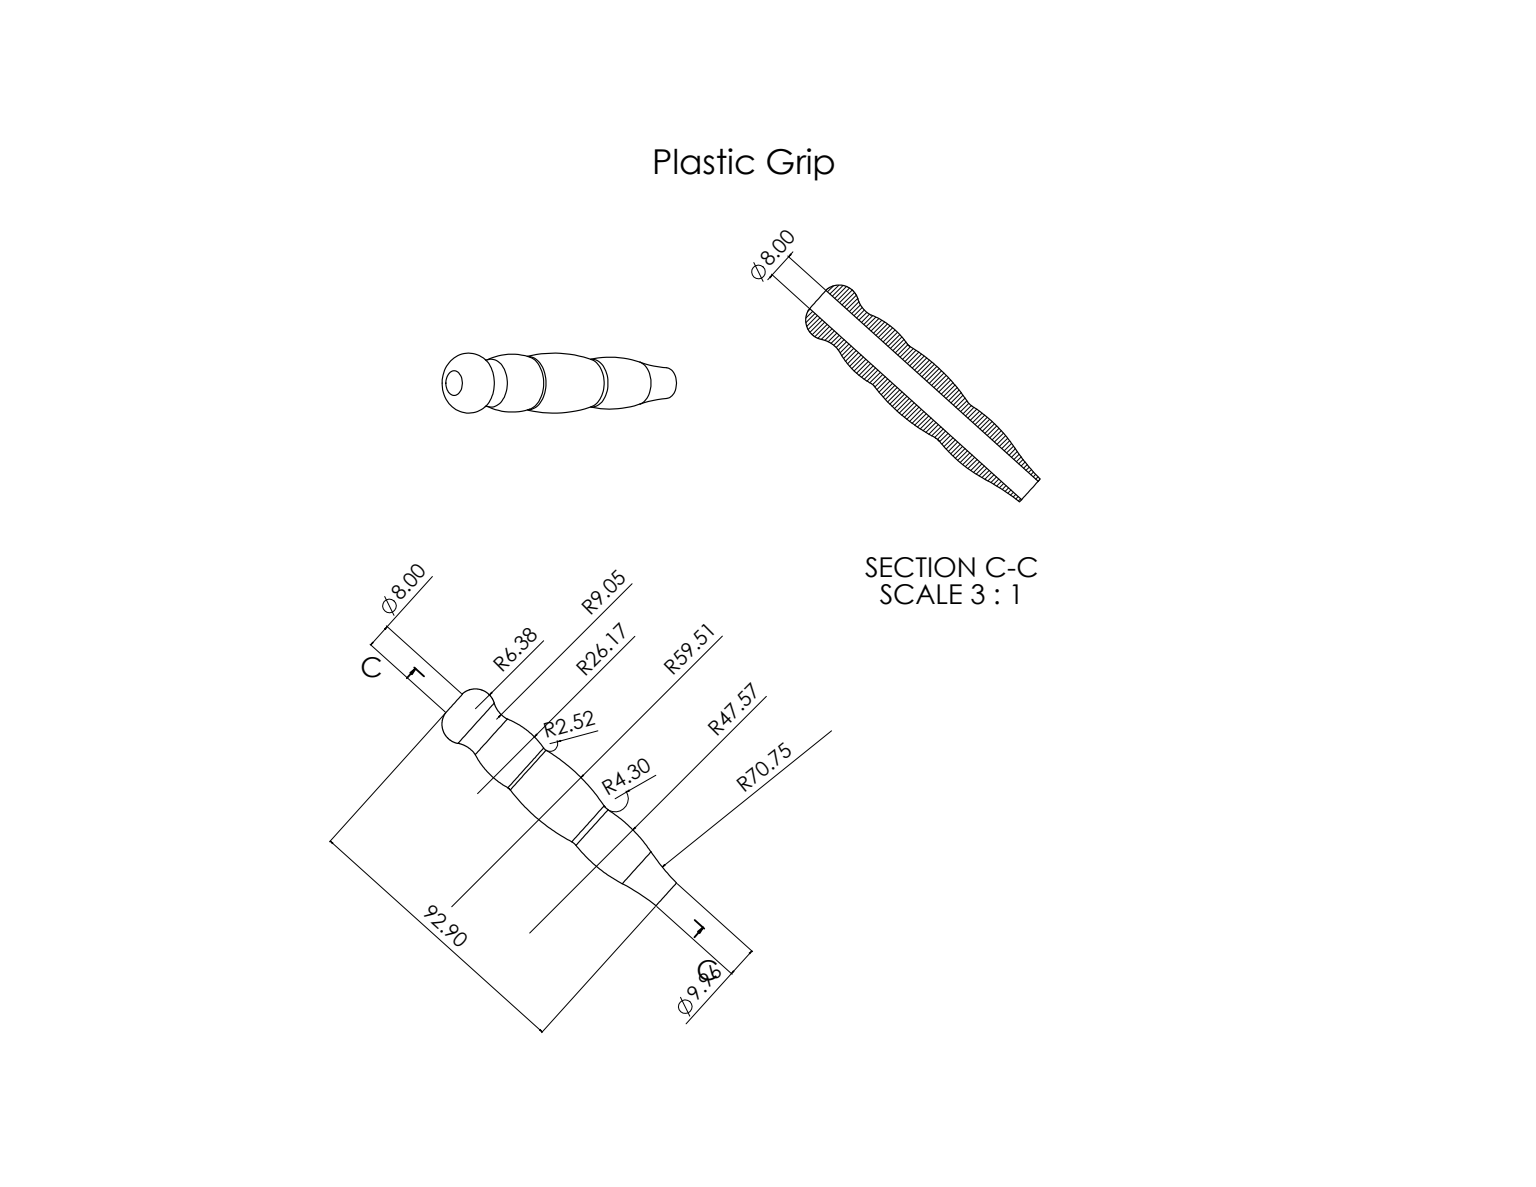
ISO-10303-21;
HEADER;
FILE_DESCRIPTION (('STEP AP214'),
    '1' );
FILE_NAME ('Plastic Grip.step',
    '2026-10-20T14:49:59',
    ( '' ),
    ( '' ),
    'SwSTEP 2.0',
    'SolidWorks 2025',
    '' );
FILE_SCHEMA (( 'AUTOMOTIVE_DESIGN' ));
ENDSEC;

DATA;
#4=DIRECTION ( 'NONE',  ( -0.6691306063588561281, -0.7431448254773960205, 0.000000000000000000 ) ) ;
#14=DIRECTION ( 'NONE',  ( -0.6691306063588562392, -0.7431448254773959095, 0.000000000000000000 ) ) ;
#16=DIRECTION ( 'NONE',  ( -0.6691306063588565722, -0.7431448254773957984, 0.000000000000000000 ) ) ;
#24=DIRECTION ( 'NONE',  ( 0.000000000000000000, -1.000000000000000000, -9.100899318238107179E-17 ) ) ;
#101=EDGE_CURVE ( 'NONE', #6753, #3816, #8421, .T. ) ;
#112=AXIS2_PLACEMENT_3D ( 'NONE', #10075, #7738, #3660 ) ;
#132=DIRECTION ( 'NONE',  ( -0.7431448254773957984, 0.6691306063588565722, -0.000000000000000000 ) ) ;
#158=CIRCLE ( 'NONE', #4883, 4.982234098198590644 ) ;
#169=EDGE_CURVE ( 'NONE', #490, #9911, #7578, .T. ) ;
#177=DIRECTION ( 'NONE',  ( -8.194486552889013533E-17, -9.100899318238110877E-17, 1.000000000000000000 ) ) ;
#179=DIRECTION ( 'NONE',  ( -0.6691306063588574604, -0.7431448254773949103, 0.000000000000000000 ) ) ;
#183=CARTESIAN_POINT ( 'NONE',  ( -147.2606667696710474, 253.8574007319445229, 0.000000000000000000 ) ) ;
#197=DIRECTION ( 'NONE',  ( -0.6691306063588565722, -0.7431448254773959095, 0.000000000000000000 ) ) ;
#213=DIRECTION ( 'NONE',  ( -0.7431448254773957984, 0.6691306063588565722, -0.000000000000000000 ) ) ;
#237=DIRECTION ( 'NONE',  ( -0.7431448254773957984, 0.6691306063588565722, -0.000000000000000000 ) ) ;
#238=ADVANCED_FACE ( 'NONE', ( #290 ), #4855, .T. ) ;
#241=CARTESIAN_POINT ( 'NONE',  ( -142.3328939341254795, 249.4204141414382434, 0.000000000000000000 ) ) ;
#247=PRODUCT_DEFINITION_FORMATION_WITH_SPECIFIED_SOURCE ( 'ANY', '', #7048, .NOT_KNOWN. ) ;
#290=FACE_OUTER_BOUND ( 'NONE', #9585, .T. ) ;
#292=AXIS2_PLACEMENT_3D ( 'NONE', #10403, #6319, #9565 ) ;
#299=DIRECTION ( 'NONE',  ( -8.194486552889013533E-17, -9.100899318238110877E-17, 1.000000000000000000 ) ) ;
#306=ORIENTED_EDGE ( 'NONE', *, *, #8464, .F. ) ;
#341=CARTESIAN_POINT ( 'NONE',  ( -152.9991366487805067, 270.9406871569508439, 1.084494555200859138E-15 ) ) ;
#347=EDGE_LOOP ( 'NONE', ( #2435, #5782, #9896, #402 ) ) ;
#357=EDGE_CURVE ( 'NONE', #2439, #4517, #2671, .T. ) ;
#394=TOROIDAL_SURFACE ( 'NONE', #3944, 11.15107097094592881, 2.515249034521771510 ) ;
#402=ORIENTED_EDGE ( 'NONE', *, *, #1707, .F. ) ;
#405=DIRECTION ( 'NONE',  ( -0.7431448254773957984, 0.6691306063588565722, -0.000000000000000000 ) ) ;
#430=EDGE_CURVE ( 'NONE', #1386, #2425, #494, .T. ) ;
#442=EDGE_LOOP ( 'NONE', ( #9473, #3806 ) ) ;
#486=ORIENTED_EDGE ( 'NONE', *, *, #169, .T. ) ;
#490=VERTEX_POINT ( 'NONE', #341 ) ;
#494=LINE ( 'NONE', #10247, #6224 ) ;
#551=TOROIDAL_SURFACE ( 'NONE', #6465, 16.62298474266377468, 9.050254677131421843 ) ;
#556=EDGE_CURVE ( 'NONE', #9911, #2425, #6732, .T. ) ;
#562=ORIENTED_EDGE ( 'NONE', *, *, #7593, .F. ) ;
#566=SHAPE_DEFINITION_REPRESENTATION ( #3920, #9697 ) ;
#576=CARTESIAN_POINT ( 'NONE',  ( -89.14744694221916177, 254.1708682956268603, 0.000000000000000000 ) ) ;
#585=ORIENTED_EDGE ( 'NONE', *, *, #5654, .F. ) ;
#591=DIRECTION ( 'NONE',  ( 0.000000000000000000, -1.000000000000000000, -9.100899318238089922E-17 ) ) ;
#594=AXIS2_PLACEMENT_3D ( 'NONE', #3166, #9596, #3115 ) ;
#617=CIRCLE ( 'NONE', #1964, 4.295524112943372330 ) ;
#642=DIRECTION ( 'NONE',  ( 0.000000000000000000, -0.000000000000000000, -1.000000000000000000 ) ) ;
#651=AXIS2_PLACEMENT_3D ( 'NONE', #10194, #3565, #8546 ) ;
#680=CARTESIAN_POINT ( 'NONE',  ( -166.0794662972351716, 270.8019239353934040, 0.000000000000000000 ) ) ;
#687=PRODUCT_DEFINITION ( 'UNKNOWN', '', #247, #5891 ) ;
#702=DIRECTION ( 'NONE',  ( -0.7431448254773957984, 0.6691306063588565722, -0.000000000000000000 ) ) ;
#728=TOROIDAL_SURFACE ( 'NONE', #9364, 3.377784142883041074, 6.382478589986769535 ) ;
#745=EDGE_CURVE ( 'NONE', #2342, #2439, #3018, .T. ) ;
#756=AXIS2_PLACEMENT_3D ( 'NONE', #4002, #6747, #591 ) ;
#765=DIRECTION ( 'NONE',  ( -0.6691306063588566833, -0.7431448254773957984, 0.000000000000000000 ) ) ;
#768=ORIENTED_EDGE ( 'NONE', *, *, #5611, .F. ) ;
#778=FACE_OUTER_BOUND ( 'NONE', #5546, .T. ) ;
#787=CIRCLE ( 'NONE', #8916, 8.635821936424155965 ) ;
#794=ORIENTED_EDGE ( 'NONE', *, *, #1876, .T. ) ;
#802=FACE_OUTER_BOUND ( 'NONE', #3369, .T. ) ;
#810=CARTESIAN_POINT ( 'NONE',  ( -142.3328939341254795, 249.4204141414382434, 0.000000000000000000 ) ) ;
#833=EDGE_CURVE ( 'NONE', #8917, #6087, #10133, .T. ) ;
#858=ORIENTED_EDGE ( 'NONE', *, *, #2768, .F. ) ;
#888=DIRECTION ( 'NONE',  ( -0.7431448254773957984, 0.6691306063588565722, -0.000000000000000000 ) ) ;
#889=AXIS2_PLACEMENT_3D ( 'NONE', #4773, #8859, #2296 ) ;
#891=CIRCLE ( 'NONE', #3260, 9.050254677131441383 ) ;
#892=DIRECTION ( 'NONE',  ( -0.7431448254773957984, 0.6691306063588565722, -0.000000000000000000 ) ) ;
#902=DIRECTION ( 'NONE',  ( -0.6691306063588566833, -0.7431448254773955764, 0.000000000000000000 ) ) ;
#961=AXIS2_PLACEMENT_3D ( 'NONE', #4774, #8012, #3991 ) ;
#1016=ORIENTED_EDGE ( 'NONE', *, *, #2108, .T. ) ;
#1025=DIRECTION ( 'NONE',  ( -0.6691306063588565722, -0.7431448254773957984, 0.000000000000000000 ) ) ;
#1052=EDGE_CURVE ( 'NONE', #9925, #6648, #8435, .T. ) ;
#1062=CARTESIAN_POINT ( 'NONE',  ( -163.4029438717997209, 273.7745032373030085, 4.898587196589436495E-16 ) ) ;
#1092=ORIENTED_EDGE ( 'NONE', *, *, #2031, .F. ) ;
#1096=AXIS2_PLACEMENT_3D ( 'NONE', #8801, #3977, #8692 ) ;
#1110=EDGE_CURVE ( 'NONE', #2425, #9911, #6741, .T. ) ;
#1124=EDGE_CURVE ( 'NONE', #4793, #490, #1337, .T. ) ;
#1138=CARTESIAN_POINT ( 'NONE',  ( -155.4728935706336301, 261.2517229562222951, 0.000000000000000000 ) ) ;
#1151=ORIENTED_EDGE ( 'NONE', *, *, #4635, .T. ) ;
#1156=DIRECTION ( 'NONE',  ( -0.7431448254773957984, 0.6691306063588565722, -0.000000000000000000 ) ) ;
#1165=CIRCLE ( 'NONE', #7936, 8.635821936424155965 ) ;
#1184=DIRECTION ( 'NONE',  ( -0.6691306063588565722, -0.7431448254773956874, 0.000000000000000000 ) ) ;
#1194=CARTESIAN_POINT ( 'NONE',  ( -117.2684580747526581, 237.4318902223653254, 9.628383344360778382E-16 ) ) ;
#1215=MECHANICAL_DESIGN_GEOMETRIC_PRESENTATION_REPRESENTATION('',(#9163),#6451);
#1241=DIRECTION ( 'NONE',  ( -8.194486552889013533E-17, -9.100899318238110877E-17, 1.000000000000000000 ) ) ;
#1246=DIRECTION ( 'NONE',  ( -0.6691306063588565722, -0.7431448254773957984, 0.000000000000000000 ) ) ;
#1259=ADVANCED_FACE ( 'NONE', ( #9754 ), #6405, .T. ) ;
#1272=ORIENTED_EDGE ( 'NONE', *, *, #10189, .T. ) ;
#1281=AXIS2_PLACEMENT_3D ( 'NONE', #3694, #405, #1246 ) ;
#1296=TOROIDAL_SURFACE ( 'NONE', #961, 12.02085523418795177, 4.295524112943378547 ) ;
#1337=CIRCLE ( 'NONE', #2348, 8.855570079111213744 ) ;
#1386=VERTEX_POINT ( 'NONE', #3486 ) ;
#1402=DIRECTION ( 'NONE',  ( -0.6691306063588565722, -0.7431448254773956874, 0.000000000000000000 ) ) ;
#1424=DIRECTION ( 'NONE',  ( -0.7431448254773957984, 0.6691306063588565722, -0.000000000000000000 ) ) ;
#1441=CIRCLE ( 'NONE', #6166, 7.794205612481196255 ) ;
#1448=DIRECTION ( 'NONE',  ( -0.7431448254773957984, 0.6691306063588565722, -0.000000000000000000 ) ) ;
#1452=AXIS2_PLACEMENT_3D ( 'NONE', #8678, #4652, #9540 ) ;
#1490=EDGE_CURVE ( 'NONE', #490, #4793, #9756, .T. ) ;
#1520=PRODUCT_CONTEXT ( 'NONE', #1525, 'mechanical' ) ;
#1525=APPLICATION_CONTEXT ( 'automotive_design' ) ;
#1531=DIRECTION ( 'NONE',  ( -0.6691306063588601249, -0.7431448254773928008, 0.000000000000000000 ) ) ;
#1544=ORIENTED_EDGE ( 'NONE', *, *, #5654, .T. ) ;
#1550=DIRECTION ( 'NONE',  ( -0.6691306063588565722, -0.7431448254773957984, 0.000000000000000000 ) ) ;
#1555=EDGE_LOOP ( 'NONE', ( #6042, #8592, #8206, #858 ) ) ;
#1573=DIRECTION ( 'NONE',  ( 0.000000000000000000, -0.000000000000000000, -1.000000000000000000 ) ) ;
#1583=CIRCLE ( 'NONE', #3443, 4.000000000000007994 ) ;
#1586=DIRECTION ( 'NONE',  ( -0.7431448254773957984, 0.6691306063588565722, -0.000000000000000000 ) ) ;
#1590=ORIENTED_EDGE ( 'NONE', *, *, #3868, .F. ) ;
#1601=DIRECTION ( 'NONE',  ( -0.7431448254773957984, 0.6691306063588565722, -0.000000000000000000 ) ) ;
#1607=ORIENTED_EDGE ( 'NONE', *, *, #3884, .T. ) ;
#1617=ORIENTED_EDGE ( 'NONE', *, *, #9294, .F. ) ;
#1620=DIRECTION ( 'NONE',  ( -0.7431448254773957984, 0.6691306063588565722, -0.000000000000000000 ) ) ;
#1629=ORIENTED_EDGE ( 'NONE', *, *, #8965, .F. ) ;
#1638=DIRECTION ( 'NONE',  ( -0.6691306063588564612, -0.7431448254773956874, 0.000000000000000000 ) ) ;
#1655=DIRECTION ( 'NONE',  ( -0.7431448254773957984, 0.6691306063588565722, -0.000000000000000000 ) ) ;
#1702=CARTESIAN_POINT ( 'NONE',  ( -142.3328939341254795, 249.4204141414382434, 0.000000000000000000 ) ) ;
#1707=EDGE_CURVE ( 'NONE', #2362, #6151, #617, .T. ) ;
#1745=ADVANCED_FACE ( 'NONE', ( #9238 ), #6205, .F. ) ;
#1754=TOROIDAL_SURFACE ( 'NONE', #7008, 75.59748767972220662, 70.74985237403969052 ) ;
#1758=DIRECTION ( 'NONE',  ( -0.7431448254773957984, 0.6691306063588565722, -0.000000000000000000 ) ) ;
#1760=AXIS2_PLACEMENT_3D ( 'NONE', #680, #3111, #2163 ) ;
#1767=DIRECTION ( 'NONE',  ( -8.194486552889013533E-17, -9.100899318238110877E-17, 1.000000000000000000 ) ) ;
#1770=ORIENTED_EDGE ( 'NONE', *, *, #1110, .T. ) ;
#1813=ORIENTED_EDGE ( 'NONE', *, *, #2108, .F. ) ;
#1818=VECTOR ( 'NONE', #8221, 1000.000000000000114 ) ;
#1821=DIRECTION ( 'NONE',  ( -0.7431448254773957984, 0.6691306063588565722, -0.000000000000000000 ) ) ;
#1822=CARTESIAN_POINT ( 'NONE',  ( -153.9940972124336156, 259.9202087346060921, 0.000000000000000000 ) ) ;
#1830=AXIS2_PLACEMENT_3D ( 'NONE', #3609, #9278, #9979 ) ;
#1839=CARTESIAN_POINT ( 'NONE',  ( -148.5890485138274357, 243.3411686721859724, 0.000000000000000000 ) ) ;
#1841=ORIENTED_EDGE ( 'NONE', *, *, #10189, .F. ) ;
#1876=EDGE_CURVE ( 'NONE', #2362, #4450, #4513, .T. ) ;
#1949=EDGE_CURVE ( 'NONE', #1386, #1994, #5353, .T. ) ;
#1951=DIRECTION ( 'NONE',  ( -0.7431448254773957984, 0.6691306063588565722, -0.000000000000000000 ) ) ;
#1964=AXIS2_PLACEMENT_3D ( 'NONE', #5307, #5253, #4469 ) ;
#1980=CARTESIAN_POINT ( 'NONE',  ( -126.4085176256957084, 224.6061440934676909, 0.000000000000000000 ) ) ;
#1994=VERTEX_POINT ( 'NONE', #10129 ) ;
#2023=ORIENTED_EDGE ( 'NONE', *, *, #6467, .F. ) ;
#2031=EDGE_CURVE ( 'NONE', #5603, #4869, #3842, .T. ) ;
#2034=CARTESIAN_POINT ( 'NONE',  ( -134.8713710537857935, 257.7072748320279061, 1.365612337163390183E-15 ) ) ;
#2039=CARTESIAN_POINT ( 'NONE',  ( -163.4029438717996641, 273.7745032373030654, 4.898587196589562712E-16 ) ) ;
#2041=CIRCLE ( 'NONE', #6279, 7.785108809001807906 ) ;
#2065=FACE_OUTER_BOUND ( 'NONE', #5158, .T. ) ;
#2075=DIRECTION ( 'NONE',  ( -0.7431448254773956874, 0.6691306063588564612, -0.000000000000000000 ) ) ;
#2080=ADVANCED_FACE ( 'NONE', ( #4069 ), #6880, .T. ) ;
#2084=CIRCLE ( 'NONE', #7345, 2.515249034521771510 ) ;
#2108=EDGE_CURVE ( 'NONE', #4793, #8917, #10105, .T. ) ;
#2135=CIRCLE ( 'NONE', #8753, 7.862171649053781408 ) ;
#2153=EDGE_CURVE ( 'NONE', #2439, #2342, #3160, .T. ) ;
#2156=ORIENTED_EDGE ( 'NONE', *, *, #5857, .T. ) ;
#2159=ORIENTED_EDGE ( 'NONE', *, *, #9094, .F. ) ;
#2163=DIRECTION ( 'NONE',  ( -0.6691306063588601249, -0.7431448254773928008, 0.000000000000000000 ) ) ;
#2176=AXIS2_PLACEMENT_3D ( 'NONE', #2955, #1586, #8257 ) ;
#2188=DIRECTION ( 'NONE',  ( -8.194486552889013533E-17, -9.100899318238110877E-17, 1.000000000000000000 ) ) ;
#2194=CARTESIAN_POINT ( 'NONE',  ( -121.7299640054770578, 230.8694527092982867, 0.000000000000000000 ) ) ;
#2209=VERTEX_POINT ( 'NONE', #5968 ) ;
#2250=CARTESIAN_POINT ( 'NONE',  ( -111.3540224549888933, 212.1074838665961124, 0.000000000000000000 ) ) ;
#2252=DIRECTION ( 'NONE',  ( -0.7431448254773957984, 0.6691306063588565722, -0.000000000000000000 ) ) ;
#2271=CYLINDRICAL_SURFACE ( 'NONE', #1760, 4.000000000000016875 ) ;
#2296=DIRECTION ( 'NONE',  ( -0.6691306063588566833, -0.7431448254773956874, 0.000000000000000000 ) ) ;
#2342=VERTEX_POINT ( 'NONE', #1839 ) ;
#2346=CARTESIAN_POINT ( 'NONE',  ( -133.6038276124207300, 241.5607275224312787, 0.000000000000000000 ) ) ;
#2348=AXIS2_PLACEMENT_3D ( 'NONE', #6563, #3221, #8145 ) ;
#2350=FACE_OUTER_BOUND ( 'NONE', #6872, .T. ) ;
#2362=VERTEX_POINT ( 'NONE', #2842 ) ;
#2379=DIRECTION ( 'NONE',  ( -0.7431448254773957984, 0.6691306063588565722, -0.000000000000000000 ) ) ;
#2425=VERTEX_POINT ( 'NONE', #6929 ) ;
#2428=CARTESIAN_POINT ( 'NONE',  ( -115.3226892516804583, 225.1003166080523954, 0.000000000000000000 ) ) ;
#2432=DIRECTION ( 'NONE',  ( -0.6691306063588580155, -0.7431448254773944662, 0.000000000000000000 ) ) ;
#2435=ORIENTED_EDGE ( 'NONE', *, *, #2550, .F. ) ;
#2439=VERTEX_POINT ( 'NONE', #5384 ) ;
#2490=TOROIDAL_SURFACE ( 'NONE', #3682, 75.59748767972220662, 70.74985237403969052 ) ;
#2539=ORIENTED_EDGE ( 'NONE', *, *, #4294, .T. ) ;
#2550=EDGE_CURVE ( 'NONE', #4450, #2362, #7596, .T. ) ;
#2604=ORIENTED_EDGE ( 'NONE', *, *, #9461, .T. ) ;
#2609=EDGE_CURVE ( 'NONE', #4517, #4542, #1165, .T. ) ;
#2650=CIRCLE ( 'NONE', #6207, 70.74985237403969052 ) ;
#2651=ORIENTED_EDGE ( 'NONE', *, *, #2153, .F. ) ;
#2671=CIRCLE ( 'NONE', #651, 2.515249034521771510 ) ;
#2703=CARTESIAN_POINT ( 'NONE',  ( -141.9789400531797412, 249.1017126355397977, 0.000000000000000000 ) ) ;
#2721=FACE_OUTER_BOUND ( 'NONE', #6822, .T. ) ;
#2724=( NAMED_UNIT ( * ) PLANE_ANGLE_UNIT ( ) SI_UNIT ( $, .RADIAN. ) );
#2733=ORIENTED_EDGE ( 'NONE', *, *, #5857, .F. ) ;
#2734=AXIS2_PLACEMENT_3D ( 'NONE', #3821, #642, #9493 ) ;
#2744=CARTESIAN_POINT ( 'NONE',  ( -126.8992195029584025, 225.1284128614458950, 0.000000000000000000 ) ) ;
#2752=CIRCLE ( 'NONE', #889, 7.785108809001807906 ) ;
#2767=FACE_OUTER_BOUND ( 'NONE', #347, .T. ) ;
#2768=EDGE_CURVE ( 'NONE', #4517, #4943, #9289, .T. ) ;
#2772=CIRCLE ( 'NONE', #8702, 26.17065043502059396 ) ;
#2779=ADVANCED_FACE ( 'NONE', ( #2721 ), #5394, .F. ) ;
#2807=EDGE_LOOP ( 'NONE', ( #1841, #3283, #8792, #3496 ) ) ;
#2829=DIRECTION ( 'NONE',  ( -0.6691306063588566833, -0.7431448254773957984, 0.000000000000000000 ) ) ;
#2839=ORIENTED_EDGE ( 'NONE', *, *, #8183, .F. ) ;
#2842=CARTESIAN_POINT ( 'NONE',  ( -116.5607085079957130, 236.6104925571506783, 9.460802029985586576E-16 ) ) ;
#2882=EDGE_CURVE ( 'NONE', #6578, #8917, #9644, .T. ) ;
#2914=AXIS2_PLACEMENT_3D ( 'NONE', #5840, #237, #4308 ) ;
#2935=DIRECTION ( 'NONE',  ( -0.7431448254773957984, 0.6691306063588565722, -0.000000000000000000 ) ) ;
#2944=EDGE_CURVE ( 'NONE', #3816, #6753, #158, .T. ) ;
#2954=FACE_OUTER_BOUND ( 'NONE', #9451, .T. ) ;
#2955=CARTESIAN_POINT ( 'NONE',  ( -166.0794662972351716, 270.8019239353934040, 0.000000000000000000 ) ) ;
#2959=FACE_OUTER_BOUND ( 'NONE', #10440, .T. ) ;
#2965=ORIENTED_EDGE ( 'NONE', *, *, #2768, .T. ) ;
#2972=DIRECTION ( 'NONE',  ( -0.6691306063588565722, -0.7431448254773957984, 0.000000000000000000 ) ) ;
#2993=ADVANCED_FACE ( 'NONE', ( #7227, #8864 ), #4926, .F. ) ;
#2999=DIRECTION ( 'NONE',  ( -0.7431448254773957984, 0.6691306063588565722, -0.000000000000000000 ) ) ;
#3009=DIRECTION ( 'NONE',  ( -1.000000000000000000, 0.000000000000000000, 0.000000000000000000 ) ) ;
#3011=ADVANCED_FACE ( 'NONE', ( #8067 ), #7604, .F. ) ;
#3018=CIRCLE ( 'NONE', #4369, 8.703944320672444945 ) ;
#3032=AXIS2_PLACEMENT_3D ( 'NONE', #810, #7276, #16 ) ;
#3053=CARTESIAN_POINT ( 'NONE',  ( -121.7299640054770578, 230.8694527092982867, 0.000000000000000000 ) ) ;
#3085=DIRECTION ( 'NONE',  ( -0.7431448254773957984, 0.6691306063588565722, -0.000000000000000000 ) ) ;
#3088=DIRECTION ( 'NONE',  ( -0.6691306063588565722, -0.7431448254773957984, 0.000000000000000000 ) ) ;
#3101=FACE_OUTER_BOUND ( 'NONE', #7591, .T. ) ;
#3111=DIRECTION ( 'NONE',  ( -0.7431448254773957984, 0.6691306063588565722, -0.000000000000000000 ) ) ;
#3115=DIRECTION ( 'NONE',  ( -0.6691306063588566833, -0.7431448254773957984, 0.000000000000000000 ) ) ;
#3125=EDGE_CURVE ( 'NONE', #4793, #2425, #7435, .T. ) ;
#3143=CARTESIAN_POINT ( 'NONE',  ( -150.4057481100919915, 266.8793581191597468, 9.273919635561124944E-16 ) ) ;
#3150=CARTESIAN_POINT ( 'NONE',  ( -160.5400390311752403, 255.6240877932848150, 0.000000000000000000 ) ) ;
#3155=ORIENTED_EDGE ( 'NONE', *, *, #2550, .T. ) ;
#3160=CIRCLE ( 'NONE', #7070, 8.703944320672444945 ) ;
#3166=CARTESIAN_POINT ( 'NONE',  ( -155.4728935706336301, 261.2517229562222951, 0.000000000000000000 ) ) ;
#3179=CARTESIAN_POINT ( 'NONE',  ( -153.9940972124336156, 259.9202087346060921, 0.000000000000000000 ) ) ;
#3184=EDGE_LOOP ( 'NONE', ( #7189, #4392, #7724, #2651 ) ) ;
#3221=DIRECTION ( 'NONE',  ( -0.7431448254773957984, 0.6691306063588565722, -0.000000000000000000 ) ) ;
#3242=AXIS2_PLACEMENT_3D ( 'NONE', #2428, #888, #5757 ) ;
#3247=DIRECTION ( 'NONE',  ( -0.6691306063588566833, -0.7431448254773957984, 0.000000000000000000 ) ) ;
#3248=CIRCLE ( 'NONE', #9348, 59.51479730733485951 ) ;
#3257=TOROIDAL_SURFACE ( 'NONE', #9703, 12.02085523418795177, 4.295524112943378547 ) ;
#3260=AXIS2_PLACEMENT_3D ( 'NONE', #8498, #299, #6697 ) ;
#3262=EDGE_LOOP ( 'NONE', ( #6618, #5581 ) ) ;
#3279=DIRECTION ( 'NONE',  ( -0.7431448254773957984, 0.6691306063588565722, -0.000000000000000000 ) ) ;
#3283=ORIENTED_EDGE ( 'NONE', *, *, #5473, .T. ) ;
#3287=ORIENTED_EDGE ( 'NONE', *, *, #3125, .F. ) ;
#3369=EDGE_LOOP ( 'NONE', ( #6942, #1272, #1590, #5013 ) ) ;
#3392=ORIENTED_EDGE ( 'NONE', *, *, #5271, .F. ) ;
#3398=AXIS2_PLACEMENT_3D ( 'NONE', #7312, #9814, #4287 ) ;
#3443=AXIS2_PLACEMENT_3D ( 'NONE', #4909, #892, #2432 ) ;
#3455=AXIS2_PLACEMENT_3D ( 'NONE', #4155, #1767, #24 ) ;
#3457=UNCERTAINTY_MEASURE_WITH_UNIT (LENGTH_MEASURE( 1.000000000000000082E-05 ), #7613, 'distance_accuracy_value', 'NONE');
#3461=ADVANCED_FACE ( 'NONE', ( #8938 ), #2490, .F. ) ;
#3466=CARTESIAN_POINT ( 'NONE',  ( -161.3589532509997468, 266.5515548974023545, 0.000000000000000000 ) ) ;
#3473=ORIENTED_EDGE ( 'NONE', *, *, #8527, .T. ) ;
#3486=CARTESIAN_POINT ( 'NONE',  ( -99.71820871057254010, 205.6674483012464520, 0.000000000000000000 ) ) ;
#3496=ORIENTED_EDGE ( 'NONE', *, *, #7879, .F. ) ;
#3500=ORIENTED_EDGE ( 'NONE', *, *, #4372, .T. ) ;
#3507=DIRECTION ( 'NONE',  ( 0.000000000000000000, -0.000000000000000000, -1.000000000000000000 ) ) ;
#3530=( LENGTH_UNIT ( ) NAMED_UNIT ( * ) SI_UNIT ( .MILLI., .METRE. ) );
#3565=DIRECTION ( 'NONE',  ( -8.194486552889013533E-17, -9.100899318238110877E-17, 1.000000000000000000 ) ) ;
#3575=DIRECTION ( 'NONE',  ( -0.7431448254773957984, 0.6691306063588565722, -0.000000000000000000 ) ) ;
#3583=ORIENTED_EDGE ( 'NONE', *, *, #745, .T. ) ;
#3609=CARTESIAN_POINT ( 'NONE',  ( -166.5958414309862690, 248.8984378607219980, 0.000000000000000000 ) ) ;
#3616=ORIENTED_EDGE ( 'NONE', *, *, #169, .F. ) ;
#3653=DIRECTION ( 'NONE',  ( -0.6691306063588566833, -0.7431448254773956874, 0.000000000000000000 ) ) ;
#3660=DIRECTION ( 'NONE',  ( -0.6691306063588580155, -0.7431448254773944662, 0.000000000000000000 ) ) ;
#3682=AXIS2_PLACEMENT_3D ( 'NONE', #4950, #1620, #197 ) ;
#3688=AXIS2_PLACEMENT_3D ( 'NONE', #2703, #5089, #4142 ) ;
#3694=CARTESIAN_POINT ( 'NONE',  ( -115.3226892516804583, 225.1003166080523954, 0.000000000000000000 ) ) ;
#3763=CARTESIAN_POINT ( 'NONE',  ( -122.5292777575814114, 231.5891580443559121, 0.000000000000000000 ) ) ;
#3798=CARTESIAN_POINT ( 'NONE',  ( -155.4728935706336301, 261.2517229562222951, 0.000000000000000000 ) ) ;
#3806=ORIENTED_EDGE ( 'NONE', *, *, #101, .F. ) ;
#3809=DIRECTION ( 'NONE',  ( -0.6691306063588565722, -0.7431448254773957984, 0.000000000000000000 ) ) ;
#3816=VERTEX_POINT ( 'NONE', #6114 ) ;
#3821=CARTESIAN_POINT ( 'NONE',  ( -129.7734861572812974, 221.9362163441986411, 0.000000000000000000 ) ) ;
#3833=CARTESIAN_POINT ( 'NONE',  ( -166.8975519277663295, 204.5843006325352746, -6.093437144708294610E-15 ) ) ;
#3842=CIRCLE ( 'NONE', #8059, 7.862171649053781408 ) ;
#3861=ORIENTED_EDGE ( 'NONE', *, *, #7879, .T. ) ;
#3866=DIRECTION ( 'NONE',  ( 0.000000000000000000, -0.000000000000000000, -1.000000000000000000 ) ) ;
#3868=EDGE_CURVE ( 'NONE', #9316, #4943, #5198, .T. ) ;
#3872=CARTESIAN_POINT ( 'NONE',  ( -113.6864418536728465, 239.8026890743979322, 1.472130188556198457E-15 ) ) ;
#3884=EDGE_CURVE ( 'NONE', #1994, #9911, #9173, .T. ) ;
#3909=EDGE_LOOP ( 'NONE', ( #3616, #7241, #7180, #9613 ) ) ;
#3916=DIRECTION ( 'NONE',  ( -1.000000000000000000, 0.000000000000000000, 0.000000000000000000 ) ) ;
#3920=PRODUCT_DEFINITION_SHAPE ( 'NONE', 'NONE',  #687 ) ;
#3933=ORIENTED_EDGE ( 'NONE', *, *, #8965, .T. ) ;
#3944=AXIS2_PLACEMENT_3D ( 'NONE', #10404, #1448, #1550 ) ;
#3977=DIRECTION ( 'NONE',  ( -0.7431448254773957984, 0.6691306063588565722, -0.000000000000000000 ) ) ;
#3991=DIRECTION ( 'NONE',  ( -0.6691306063588565722, -0.7431448254773956874, 0.000000000000000000 ) ) ;
#4002=CARTESIAN_POINT ( 'NONE',  ( -144.3499457102809913, 273.6050080517225638, 2.035728505737848743E-15 ) ) ;
#4069=FACE_OUTER_BOUND ( 'NONE', #2807, .T. ) ;
#4142=DIRECTION ( 'NONE',  ( -0.6691306063588549069, -0.7431448254773971307, 0.000000000000000000 ) ) ;
#4146=CARTESIAN_POINT ( 'NONE',  ( -93.70792096198771048, 212.3425490925493762, 0.000000000000000000 ) ) ;
#4155=CARTESIAN_POINT ( 'NONE',  ( -158.4738950245593117, 241.4038491004292837, -2.052251677020569255E-15 ) ) ;
#4201=AXIS2_PLACEMENT_3D ( 'NONE', #6196, #5452, #4606 ) ;
#4258=FACE_OUTER_BOUND ( 'NONE', #1555, .T. ) ;
#4260=AXIS2_PLACEMENT_3D ( 'NONE', #2194, #6219, #1402 ) ;
#4287=DIRECTION ( 'NONE',  ( -1.000000000000000000, 0.000000000000000000, 0.000000000000000000 ) ) ;
#4294=EDGE_CURVE ( 'NONE', #2342, #4542, #5981, .T. ) ;
#4298=ORIENTED_EDGE ( 'NONE', *, *, #1052, .T. ) ;
#4302=CARTESIAN_POINT ( 'NONE',  ( -163.6191320026764231, 264.0413720900392036, 0.000000000000000000 ) ) ;
#4304=ORIENTED_EDGE ( 'NONE', *, *, #5557, .T. ) ;
#4308=DIRECTION ( 'NONE',  ( -0.6691306063588562392, -0.7431448254773960205, 0.000000000000000000 ) ) ;
#4352=EDGE_LOOP ( 'NONE', ( #2539, #4304, #8852, #4892 ) ) ;
#4358=AXIS2_PLACEMENT_3D ( 'NONE', #3872, #8887, #7837 ) ;
#4369=AXIS2_PLACEMENT_3D ( 'NONE', #4872, #6622, #902 ) ;
#4372=EDGE_CURVE ( 'NONE', #8917, #6578, #5664, .T. ) ;
#4391=AXIS2_PLACEMENT_3D ( 'NONE', #2034, #1241, #8499 ) ;
#4392=ORIENTED_EDGE ( 'NONE', *, *, #2609, .T. ) ;
#4410=ORIENTED_EDGE ( 'NONE', *, *, #9461, .F. ) ;
#4450=VERTEX_POINT ( 'NONE', #2744 ) ;
#4469=DIRECTION ( 'NONE',  ( 0.000000000000000000, -1.000000000000000000, -9.100899318238123202E-17 ) ) ;
#4490=ORIENTED_EDGE ( 'NONE', *, *, #2882, .T. ) ;
#4496=CARTESIAN_POINT ( 'NONE',  ( -148.1113867028520872, 243.0027477556404563, 0.000000000000000000 ) ) ;
#4500=DIRECTION ( 'NONE',  ( -0.6691306063588562392, -0.7431448254773959095, 0.000000000000000000 ) ) ;
#4509=DIRECTION ( 'NONE',  ( -0.7431448254773957984, 0.6691306063588565722, -0.000000000000000000 ) ) ;
#4513=CIRCLE ( 'NONE', #292, 7.725331121244574994 ) ;
#4517=VERTEX_POINT ( 'NONE', #8419 ) ;
#4522=DIRECTION ( 'NONE',  ( -0.7431448254773957984, 0.6691306063588565722, -0.000000000000000000 ) ) ;
#4542=VERTEX_POINT ( 'NONE', #4496 ) ;
#4545=CARTESIAN_POINT ( 'NONE',  ( -155.4728935706336301, 261.2517229562222951, 0.000000000000000000 ) ) ;
#4558=DIRECTION ( 'NONE',  ( -0.7431448254773957984, 0.6691306063588565722, -0.000000000000000000 ) ) ;
#4590=ADVANCED_FACE ( 'NONE', ( #5495 ), #10281, .F. ) ;
#4596=CARTESIAN_POINT ( 'NONE',  ( -149.7944168144651655, 241.1335534508485807, 0.000000000000000000 ) ) ;
#4599=CARTESIAN_POINT ( 'NONE',  ( -141.4979315611417690, 196.0297649204779589, -4.790608351577442020E-15 ) ) ;
#4601=AXIS2_PLACEMENT_3D ( 'NONE', #8586, #5983, #5928 ) ;
#4606=DIRECTION ( 'NONE',  ( -0.6691306063588562392, -0.7431448254773960205, 0.000000000000000000 ) ) ;
#4635=EDGE_CURVE ( 'NONE', #9925, #6753, #10417, .T. ) ;
#4648=CARTESIAN_POINT ( 'NONE',  ( -158.9246696254695337, 264.3597160760069187, 0.000000000000000000 ) ) ;
#4652=DIRECTION ( 'NONE',  ( -8.194486552889013533E-17, -9.100899318238110877E-17, 1.000000000000000000 ) ) ;
#4681=CIRCLE ( 'NONE', #5852, 7.794205612481196255 ) ;
#4729=ORIENTED_EDGE ( 'NONE', *, *, #9294, .T. ) ;
#4739=DIRECTION ( 'NONE',  ( -0.7431448254773957984, 0.6691306063588565722, -0.000000000000000000 ) ) ;
#4753=ORIENTED_EDGE ( 'NONE', *, *, #1110, .F. ) ;
#4770=DIRECTION ( 'NONE',  ( 0.000000000000000000, -1.000000000000000000, -9.100899318238112109E-17 ) ) ;
#4773=CARTESIAN_POINT ( 'NONE',  ( -121.1992630477586346, 230.3916074206559017, 0.000000000000000000 ) ) ;
#4774=CARTESIAN_POINT ( 'NONE',  ( -121.7299640054770578, 230.8694527092982867, 0.000000000000000000 ) ) ;
#4793=VERTEX_POINT ( 'NONE', #9744 ) ;
#4803=TOROIDAL_SURFACE ( 'NONE', #6163, 11.15107097094592881, 2.515249034521771510 ) ;
#4845=ORIENTED_EDGE ( 'NONE', *, *, #1124, .T. ) ;
#4855=TOROIDAL_SURFACE ( 'NONE', #6220, -16.75790667520975674, 26.17065043502059041 ) ;
#4856=CARTESIAN_POINT ( 'NONE',  ( -166.5958414309862690, 248.8984378607219980, 0.000000000000000000 ) ) ;
#4869=VERTEX_POINT ( 'NONE', #1194 ) ;
#4872=CARTESIAN_POINT ( 'NONE',  ( -142.7649729728221359, 249.8094598553370531, 0.000000000000000000 ) ) ;
#4881=ADVANCED_FACE ( 'NONE', ( #7661 ), #9760, .T. ) ;
#4882=ORIENTED_EDGE ( 'NONE', *, *, #430, .T. ) ;
#4883=AXIS2_PLACEMENT_3D ( 'NONE', #9831, #1758, #179 ) ;
#4892=ORIENTED_EDGE ( 'NONE', *, *, #745, .F. ) ;
#4909=CARTESIAN_POINT ( 'NONE',  ( -97.04168628513710360, 208.6400276031560281, 0.000000000000000000 ) ) ;
#4926=PLANE ( 'NONE',  #9120 ) ;
#4943=VERTEX_POINT ( 'NONE', #9633 ) ;
#4950=CARTESIAN_POINT ( 'NONE',  ( -93.80004353141508489, 205.7212393575359783, 0.000000000000000000 ) ) ;
#4953=CIRCLE ( 'NONE', #5292, 8.681329343575942659 ) ;
#4967=CARTESIAN_POINT ( 'NONE',  ( -155.4728935706336301, 261.2517229562222951, 0.000000000000000000 ) ) ;
#4975=CIRCLE ( 'NONE', #3455, 26.17065043502059396 ) ;
#4979=ORIENTED_EDGE ( 'NONE', *, *, #9094, .T. ) ;
#5013=ORIENTED_EDGE ( 'NONE', *, *, #7178, .F. ) ;
#5052=AXIS2_PLACEMENT_3D ( 'NONE', #1138, #3575, #6111 ) ;
#5089=DIRECTION ( 'NONE',  ( -0.7431448254773957984, 0.6691306063588565722, -0.000000000000000000 ) ) ;
#5158=EDGE_LOOP ( 'NONE', ( #4845, #486, #4753, #3287 ) ) ;
#5168=ORIENTED_EDGE ( 'NONE', *, *, #1949, .F. ) ;
#5198=CIRCLE ( 'NONE', #3688, 8.681329343575942659 ) ;
#5240=ORIENTED_EDGE ( 'NONE', *, *, #5611, .T. ) ;
#5253=DIRECTION ( 'NONE',  ( -8.194486552889013533E-17, -9.100899318238110877E-17, 1.000000000000000000 ) ) ;
#5255=DIRECTION ( 'NONE',  ( -0.7431448254773957984, 0.6691306063588565722, -0.000000000000000000 ) ) ;
#5262=TOROIDAL_SURFACE ( 'NONE', #4260, 12.02085523418795177, 4.295524112943378547 ) ;
#5271=EDGE_CURVE ( 'NONE', #2209, #6087, #4681, .T. ) ;
#5292=AXIS2_PLACEMENT_3D ( 'NONE', #6949, #4558, #6038 ) ;
#5293=ORIENTED_EDGE ( 'NONE', *, *, #9517, .F. ) ;
#5295=CIRCLE ( 'NONE', #4358, 4.295524112943372330 ) ;
#5307=CARTESIAN_POINT ( 'NONE',  ( -113.6864418536728465, 239.8026890743979322, 1.472130188556198457E-15 ) ) ;
#5313=TOROIDAL_SURFACE ( 'NONE', #5650, 3.377784142883041074, 6.382478589986769535 ) ;
#5318=CIRCLE ( 'NONE', #756, 9.050254677131441383 ) ;
#5333=CARTESIAN_POINT ( 'NONE',  ( -100.3101032970751305, 278.5371544123273111, 0.000000000000000000 ) ) ;
#5353=CIRCLE ( 'NONE', #112, 4.000000000000007994 ) ;
#5372=ORIENTED_EDGE ( 'NONE', *, *, #556, .T. ) ;
#5384=CARTESIAN_POINT ( 'NONE',  ( -136.9408974318168646, 256.2777510384881339, 1.065925755226830171E-15 ) ) ;
#5394=TOROIDAL_SURFACE ( 'NONE', #8783, 16.62298474266377468, 9.050254677131421843 ) ;
#5414=CARTESIAN_POINT ( 'NONE',  ( -166.0794662972351716, 270.8019239353934040, 0.000000000000000000 ) ) ;
#5452=DIRECTION ( 'NONE',  ( -0.7431448254773957984, 0.6691306063588565722, -0.000000000000000000 ) ) ;
#5473=EDGE_CURVE ( 'NONE', #4869, #5603, #2135, .T. ) ;
#5477=DIRECTION ( 'NONE',  ( -0.6691306063588574604, -0.7431448254773949103, 0.000000000000000000 ) ) ;
#5495=FACE_OUTER_BOUND ( 'NONE', #9273, .T. ) ;
#5502=DIRECTION ( 'NONE',  ( -0.6691306063588566833, -0.7431448254773955764, 0.000000000000000000 ) ) ;
#5519=FACE_OUTER_BOUND ( 'NONE', #4352, .T. ) ;
#5537=AXIS2_PLACEMENT_3D ( 'NONE', #7080, #7230, #6330 ) ;
#5545=CARTESIAN_POINT ( 'NONE',  ( -142.3328939341254795, 249.4204141414382434, 0.000000000000000000 ) ) ;
#5546=EDGE_LOOP ( 'NONE', ( #5571, #4979, #8645, #9724 ) ) ;
#5549=DIRECTION ( 'NONE',  ( -0.7431448254773957984, 0.6691306063588565722, -0.000000000000000000 ) ) ;
#5557=EDGE_CURVE ( 'NONE', #4542, #4517, #787, .T. ) ;
#5571=ORIENTED_EDGE ( 'NONE', *, *, #2882, .F. ) ;
#5581=ORIENTED_EDGE ( 'NONE', *, *, #8183, .T. ) ;
#5582=CARTESIAN_POINT ( 'NONE',  ( -97.04168628513711781, 208.6400276031560566, 0.000000000000000000 ) ) ;
#5584=ADVANCED_FACE ( 'NONE', ( #8809 ), #1296, .F. ) ;
#5591=ORIENTED_EDGE ( 'NONE', *, *, #3884, .F. ) ;
#5603=VERTEX_POINT ( 'NONE', #7638 ) ;
#5611=EDGE_CURVE ( 'NONE', #9925, #6151, #7564, .T. ) ;
#5650=AXIS2_PLACEMENT_3D ( 'NONE', #3466, #7495, #1025 ) ;
#5654=EDGE_CURVE ( 'NONE', #6648, #3816, #2650, .T. ) ;
#5663=ORIENTED_EDGE ( 'NONE', *, *, #1490, .F. ) ;
#5664=CIRCLE ( 'NONE', #8720, 7.572730065532343069 ) ;
#5712=ORIENTED_EDGE ( 'NONE', *, *, #1052, .F. ) ;
#5757=DIRECTION ( 'NONE',  ( -0.6691306063588565722, -0.7431448254773957984, 0.000000000000000000 ) ) ;
#5759=FACE_OUTER_BOUND ( 'NONE', #9367, .T. ) ;
#5779=AXIS2_PLACEMENT_3D ( 'NONE', #3833, #2188, #4770 ) ;
#5782=ORIENTED_EDGE ( 'NONE', *, *, #6775, .T. ) ;
#5802=ADVANCED_FACE ( 'NONE', ( #778 ), #8025, .F. ) ;
#5822=ORIENTED_EDGE ( 'NONE', *, *, #4635, .F. ) ;
#5840=CARTESIAN_POINT ( 'NONE',  ( -106.6701082104768687, 217.3094976449379203, 0.000000000000000000 ) ) ;
#5852=AXIS2_PLACEMENT_3D ( 'NONE', #1822, #5255, #9241 ) ;
#5857=EDGE_CURVE ( 'NONE', #4869, #2362, #5295, .T. ) ;
#5869=DIRECTION ( 'NONE',  ( -1.000000000000000000, 0.000000000000000000, 0.000000000000000000 ) ) ;
#5891=PRODUCT_DEFINITION_CONTEXT ( 'detailed design', #10047, 'design' ) ;
#5928=DIRECTION ( 'NONE',  ( 1.000000000000000000, 0.000000000000000000, 0.000000000000000000 ) ) ;
#5932=CIRCLE ( 'NONE', #3398, 4.295524112943372330 ) ;
#5934=DIRECTION ( 'NONE',  ( -1.000000000000000000, 0.000000000000000000, 0.000000000000000000 ) ) ;
#5953=TOROIDAL_SURFACE ( 'NONE', #10032, 16.62298474266377468, 9.050254677131421843 ) ;
#5960=ORIENTED_EDGE ( 'NONE', *, *, #1707, .T. ) ;
#5968=CARTESIAN_POINT ( 'NONE',  ( -148.7787556848684858, 265.7124323042283436, 9.545148955221437884E-16 ) ) ;
#5981=CIRCLE ( 'NONE', #10413, 2.515249034521771510 ) ;
#5983=DIRECTION ( 'NONE',  ( 0.000000000000000000, 0.000000000000000000, 1.000000000000000000 ) ) ;
#5997=DIRECTION ( 'NONE',  ( -0.7431448254773957984, 0.6691306063588565722, -0.000000000000000000 ) ) ;
#6000=TOROIDAL_SURFACE ( 'NONE', #1096, 11.15107097094592881, 2.515249034521771510 ) ;
#6021=DIRECTION ( 'NONE',  ( -0.6691306063588564612, -0.7431448254773957984, 0.000000000000000000 ) ) ;
#6038=DIRECTION ( 'NONE',  ( -0.6691306063588549069, -0.7431448254773971307, 0.000000000000000000 ) ) ;
#6042=ORIENTED_EDGE ( 'NONE', *, *, #5557, .F. ) ;
#6047=ORIENTED_EDGE ( 'NONE', *, *, #7593, .T. ) ;
#6074=AXIS2_PLACEMENT_3D ( 'NONE', #4302, #8147, #9107 ) ;
#6087=VERTEX_POINT ( 'NONE', #9313 ) ;
#6111=DIRECTION ( 'NONE',  ( -0.6691306063588564612, -0.7431448254773956874, 0.000000000000000000 ) ) ;
#6114=CARTESIAN_POINT ( 'NONE',  ( -100.3754516082865393, 204.9375061137627370, 0.000000000000000000 ) ) ;
#6151=VERTEX_POINT ( 'NONE', #6385 ) ;
#6158=CARTESIAN_POINT ( 'NONE',  ( -121.7299640054770578, 230.8694527092982867, 0.000000000000000000 ) ) ;
#6163=AXIS2_PLACEMENT_3D ( 'NONE', #241, #1821, #2972 ) ;
#6166=AXIS2_PLACEMENT_3D ( 'NONE', #3179, #2379, #4 ) ;
#6196=CARTESIAN_POINT ( 'NONE',  ( -106.6701082104768687, 217.3094976449379203, 0.000000000000000000 ) ) ;
#6205=TOROIDAL_SURFACE ( 'NONE', #6710, 12.02085523418795177, 4.295524112943378547 ) ;
#6207=AXIS2_PLACEMENT_3D ( 'NONE', #9433, #3507, #5934 ) ;
#6219=DIRECTION ( 'NONE',  ( -0.7431448254773957984, 0.6691306063588565722, -0.000000000000000000 ) ) ;
#6220=AXIS2_PLACEMENT_3D ( 'NONE', #183, #132, #6638 ) ;
#6224=VECTOR ( 'NONE', #2075, 1000.000000000000114 ) ;
#6247=ADVANCED_FACE ( 'NONE', ( #3101 ), #551, .F. ) ;
#6265=DIRECTION ( 'NONE',  ( -0.6691306063588601249, -0.7431448254773928008, 0.000000000000000000 ) ) ;
#6279=AXIS2_PLACEMENT_3D ( 'NONE', #10125, #1951, #3653 ) ;
#6282=DIRECTION ( 'NONE',  ( -0.7431448254773957984, 0.6691306063588565722, -0.000000000000000000 ) ) ;
#6287=DIRECTION ( 'NONE',  ( -0.6691306063588547959, -0.7431448254773973527, 0.000000000000000000 ) ) ;
#6288=DIRECTION ( 'NONE',  ( -0.7431448254773957984, 0.6691306063588565722, -0.000000000000000000 ) ) ;
#6298=CARTESIAN_POINT ( 'NONE',  ( -142.7649729728221359, 249.8094598553370531, 0.000000000000000000 ) ) ;
#6319=DIRECTION ( 'NONE',  ( -0.7431448254773957984, 0.6691306063588565722, -0.000000000000000000 ) ) ;
#6330=DIRECTION ( 'NONE',  ( 0.000000000000000000, -1.000000000000000000, -9.100899318238137994E-17 ) ) ;
#6385=CARTESIAN_POINT ( 'NONE',  ( -115.9900084698215608, 236.1770707478440841, 9.534008583957946635E-16 ) ) ;
#6400=CARTESIAN_POINT ( 'NONE',  ( -133.6038276124207300, 241.5607275224312787, 0.000000000000000000 ) ) ;
#6405=TOROIDAL_SURFACE ( 'NONE', #7764, -16.75790667520975674, 26.17065043502059041 ) ;
#6451=( GEOMETRIC_REPRESENTATION_CONTEXT ( 3 ) GLOBAL_UNCERTAINTY_ASSIGNED_CONTEXT ( ( #3457 ) ) GLOBAL_UNIT_ASSIGNED_CONTEXT ( ( #7613, #7561, #10106 ) ) REPRESENTATION_CONTEXT ( 'NONE', 'WORKASPACE' ) );
#6465=AXIS2_PLACEMENT_3D ( 'NONE', #3798, #2999, #765 ) ;
#6467=EDGE_CURVE ( 'NONE', #490, #6578, #891, .T. ) ;
#6480=DIRECTION ( 'NONE',  ( 0.000000000000000000, -0.000000000000000000, -1.000000000000000000 ) ) ;
#6524=VERTEX_POINT ( 'NONE', #1980 ) ;
#6563=CARTESIAN_POINT ( 'NONE',  ( -158.9246696254695337, 264.3597160760069187, 0.000000000000000000 ) ) ;
#6578=VERTEX_POINT ( 'NONE', #3143 ) ;
#6618=ORIENTED_EDGE ( 'NONE', *, *, #1949, .T. ) ;
#6622=DIRECTION ( 'NONE',  ( -0.7431448254773957984, 0.6691306063588565722, -0.000000000000000000 ) ) ;
#6638=DIRECTION ( 'NONE',  ( -0.6691306063588564612, -0.7431448254773957984, 0.000000000000000000 ) ) ;
#6648=VERTEX_POINT ( 'NONE', #2250 ) ;
#6697=DIRECTION ( 'NONE',  ( 0.000000000000000000, -1.000000000000000000, -9.100899318238089922E-17 ) ) ;
#6702=ADVANCED_FACE ( 'NONE', ( #2350 ), #5262, .F. ) ;
#6706=( NAMED_UNIT ( * ) SI_UNIT ( $, .STERADIAN. ) SOLID_ANGLE_UNIT ( ) );
#6710=AXIS2_PLACEMENT_3D ( 'NONE', #6909, #5997, #7646 ) ;
#6732=CIRCLE ( 'NONE', #8254, 4.000000000000016875 ) ;
#6741=CIRCLE ( 'NONE', #2176, 4.000000000000016875 ) ;
#6747=DIRECTION ( 'NONE',  ( -8.194486552889013533E-17, -9.100899318238110877E-17, 1.000000000000000000 ) ) ;
#6750=ORIENTED_EDGE ( 'NONE', *, *, #5473, .F. ) ;
#6753=VERTEX_POINT ( 'NONE', #8796 ) ;
#6756=SHAPE_REPRESENTATION_RELATIONSHIP ( 'NONE' , 'NONE' ,  #9697, #9745 ) ;
#6775=EDGE_CURVE ( 'NONE', #4450, #6524, #6799, .T. ) ;
#6799=CIRCLE ( 'NONE', #2734, 4.295524112943372330 ) ;
#6814=TOROIDAL_SURFACE ( 'NONE', #9541, -49.75669024694125397, 59.51479730733485951 ) ;
#6822=EDGE_LOOP ( 'NONE', ( #1016, #3500, #2023, #8555 ) ) ;
#6837=ADVANCED_FACE ( 'NONE', ( #9440 ), #7814, .T. ) ;
#6872=EDGE_LOOP ( 'NONE', ( #8288, #5960, #6047, #7479 ) ) ;
#6880=TOROIDAL_SURFACE ( 'NONE', #9602, -49.75669024694125397, 59.51479730733485951 ) ;
#6909=CARTESIAN_POINT ( 'NONE',  ( -121.7299640054770578, 230.8694527092982867, 0.000000000000000000 ) ) ;
#6929=CARTESIAN_POINT ( 'NONE',  ( -168.7559887226705087, 267.8293446334839700, 0.000000000000000000 ) ) ;
#6934=CARTESIAN_POINT ( 'NONE',  ( -147.2606667696710474, 253.8574007319445229, 0.000000000000000000 ) ) ;
#6942=ORIENTED_EDGE ( 'NONE', *, *, #2031, .T. ) ;
#6949=CARTESIAN_POINT ( 'NONE',  ( -141.9789400531797412, 249.1017126355397977, 0.000000000000000000 ) ) ;
#7008=AXIS2_PLACEMENT_3D ( 'NONE', #9054, #3279, #7308 ) ;
#7034=ORIENTED_EDGE ( 'NONE', *, *, #2609, .F. ) ;
#7048=PRODUCT ( 'Plastic Grip', 'Plastic Grip', '', ( #1520 ) ) ;
#7060=CARTESIAN_POINT ( 'NONE',  ( -147.7878832208476183, 242.6502276555962396, 0.000000000000000000 ) ) ;
#7070=AXIS2_PLACEMENT_3D ( 'NONE', #6298, #10438, #5502 ) ;
#7077=AXIS2_PLACEMENT_3D ( 'NONE', #5582, #2252, #5477 ) ;
#7080=CARTESIAN_POINT ( 'NONE',  ( -159.0987744993230706, 269.0617377047655054, 4.136592538792403018E-16 ) ) ;
#7091=DIRECTION ( 'NONE',  ( -0.6691306063588553510, -0.7431448254773969087, 0.000000000000000000 ) ) ;
#7101=CARTESIAN_POINT ( 'NONE',  ( -166.0794662972351716, 270.8019239353934040, 0.000000000000000000 ) ) ;
#7167=ADVANCED_FACE ( 'NONE', ( #2954 ), #5953, .F. ) ;
#7178=EDGE_CURVE ( 'NONE', #5603, #9316, #3248, .T. ) ;
#7180=ORIENTED_EDGE ( 'NONE', *, *, #3125, .T. ) ;
#7189=ORIENTED_EDGE ( 'NONE', *, *, #357, .T. ) ;
#7198=DIRECTION ( 'NONE',  ( -1.000000000000000000, 0.000000000000000000, 0.000000000000000000 ) ) ;
#7216=EDGE_LOOP ( 'NONE', ( #7034, #2965, #3861, #306 ) ) ;
#7227=FACE_OUTER_BOUND ( 'NONE', #442, .T. ) ;
#7230=DIRECTION ( 'NONE',  ( -8.194486552889013533E-17, -9.100899318238110877E-17, 1.000000000000000000 ) ) ;
#7236=CLOSED_SHELL ( 'NONE', ( #1745, #7616, #2779, #7167, #3011, #5584, #4590, #8245, #4881, #6702, #7607, #9277, #1259, #5802, #7918, #9095, #6247, #238, #9111, #2080, #7410, #6837, #3461, #2993, #8538 ) ) ;
#7237=ORIENTED_EDGE ( 'NONE', *, *, #7301, .F. ) ;
#7241=ORIENTED_EDGE ( 'NONE', *, *, #1490, .T. ) ;
#7276=DIRECTION ( 'NONE',  ( -0.7431448254773957984, 0.6691306063588565722, -0.000000000000000000 ) ) ;
#7301=EDGE_CURVE ( 'NONE', #6648, #9925, #7486, .T. ) ;
#7308=DIRECTION ( 'NONE',  ( -0.6691306063588565722, -0.7431448254773959095, 0.000000000000000000 ) ) ;
#7312=CARTESIAN_POINT ( 'NONE',  ( -129.7734861572812974, 221.9362163441986411, 0.000000000000000000 ) ) ;
#7345=AXIS2_PLACEMENT_3D ( 'NONE', #4596, #1573, #7198 ) ;
#7354=ORIENTED_EDGE ( 'NONE', *, *, #833, .T. ) ;
#7410=ADVANCED_FACE ( 'NONE', ( #2767 ), #3257, .F. ) ;
#7432=DIRECTION ( 'NONE',  ( -0.6691306063588560171, -0.7431448254773961315, 0.000000000000000000 ) ) ;
#7433=ORIENTED_EDGE ( 'NONE', *, *, #7301, .T. ) ;
#7435=CIRCLE ( 'NONE', #6074, 6.382478589986778417 ) ;
#7479=ORIENTED_EDGE ( 'NONE', *, *, #6775, .F. ) ;
#7486=CIRCLE ( 'NONE', #2914, 7.000000000000016875 ) ;
#7495=DIRECTION ( 'NONE',  ( -0.7431448254773957984, 0.6691306063588565722, -0.000000000000000000 ) ) ;
#7561=( NAMED_UNIT ( * ) PLANE_ANGLE_UNIT ( ) SI_UNIT ( $, .RADIAN. ) );
#7564=CIRCLE ( 'NONE', #8241, 47.56532671630425568 ) ;
#7578=CIRCLE ( 'NONE', #5537, 6.382478589986750883 ) ;
#7586=CARTESIAN_POINT ( 'NONE',  ( -161.3589532509997468, 266.5515548974023545, 0.000000000000000000 ) ) ;
#7591=EDGE_LOOP ( 'NONE', ( #9394, #7354, #4729, #2159 ) ) ;
#7593=EDGE_CURVE ( 'NONE', #6151, #6524, #2752, .T. ) ;
#7596=CIRCLE ( 'NONE', #8946, 7.725331121244574994 ) ;
#7604=TOROIDAL_SURFACE ( 'NONE', #3032, 11.15107097094592881, 2.515249034521771510 ) ;
#7607=ADVANCED_FACE ( 'NONE', ( #802 ), #6814, .T. ) ;
#7613=( LENGTH_UNIT ( ) NAMED_UNIT ( * ) SI_UNIT ( .MILLI., .METRE. ) );
#7616=ADVANCED_FACE ( 'NONE', ( #5519 ), #394, .F. ) ;
#7638=CARTESIAN_POINT ( 'NONE',  ( -127.7900974404101930, 225.7464258663465557, 0.000000000000000000 ) ) ;
#7646=DIRECTION ( 'NONE',  ( -0.6691306063588565722, -0.7431448254773956874, 0.000000000000000000 ) ) ;
#7661=FACE_OUTER_BOUND ( 'NONE', #10437, .T. ) ;
#7683=CIRCLE ( 'NONE', #8531, 47.56532671630425568 ) ;
#7696=ORIENTED_EDGE ( 'NONE', *, *, #8449, .T. ) ;
#7724=ORIENTED_EDGE ( 'NONE', *, *, #4294, .F. ) ;
#7738=DIRECTION ( 'NONE',  ( -0.7431448254773957984, 0.6691306063588565722, -0.000000000000000000 ) ) ;
#7764=AXIS2_PLACEMENT_3D ( 'NONE', #6934, #1156, #6021 ) ;
#7814=TOROIDAL_SURFACE ( 'NONE', #3242, -39.11828581851394659, 47.56532671630426989 ) ;
#7837=DIRECTION ( 'NONE',  ( 0.000000000000000000, -1.000000000000000000, -9.100899318238123202E-17 ) ) ;
#7879=EDGE_CURVE ( 'NONE', #4943, #9316, #4953, .T. ) ;
#7918=ADVANCED_FACE ( 'NONE', ( #2065 ), #728, .T. ) ;
#7934=DIRECTION ( 'NONE',  ( -0.6691306063588560171, -0.7431448254773961315, 0.000000000000000000 ) ) ;
#7936=AXIS2_PLACEMENT_3D ( 'NONE', #5545, #4739, #7934 ) ;
#7940=DIRECTION ( 'NONE',  ( -1.000000000000000000, 0.000000000000000000, 0.000000000000000000 ) ) ;
#8012=DIRECTION ( 'NONE',  ( -0.7431448254773957984, 0.6691306063588565722, -0.000000000000000000 ) ) ;
#8025=TOROIDAL_SURFACE ( 'NONE', #594, 16.62298474266377468, 9.050254677131421843 ) ;
#8059=AXIS2_PLACEMENT_3D ( 'NONE', #3763, #9382, #4500 ) ;
#8067=FACE_OUTER_BOUND ( 'NONE', #3184, .T. ) ;
#8132=EDGE_LOOP ( 'NONE', ( #2156, #794, #4410, #6750 ) ) ;
#8142=DIRECTION ( 'NONE',  ( -0.7431448254773957984, 0.6691306063588565722, -0.000000000000000000 ) ) ;
#8145=DIRECTION ( 'NONE',  ( -0.6691306063588547959, -0.7431448254773973527, 0.000000000000000000 ) ) ;
#8147=DIRECTION ( 'NONE',  ( 0.000000000000000000, -0.000000000000000000, -1.000000000000000000 ) ) ;
#8149=CARTESIAN_POINT ( 'NONE',  ( -149.7944168144651655, 241.1335534508485807, 0.000000000000000000 ) ) ;
#8170=DIRECTION ( 'NONE',  ( -0.7431448254773957984, 0.6691306063588565722, 0.000000000000000000 ) ) ;
#8183=EDGE_CURVE ( 'NONE', #1994, #1386, #1583, .T. ) ;
#8206=ORIENTED_EDGE ( 'NONE', *, *, #3868, .T. ) ;
#8221=DIRECTION ( 'NONE',  ( -0.7431448254773956874, 0.6691306063588564612, -0.000000000000000000 ) ) ;
#8241=AXIS2_PLACEMENT_3D ( 'NONE', #4599, #177, #9229 ) ;
#8245=ADVANCED_FACE ( 'NONE', ( #5759 ), #1754, .F. ) ;
#8254=AXIS2_PLACEMENT_3D ( 'NONE', #5414, #3085, #6265 ) ;
#8257=DIRECTION ( 'NONE',  ( -0.6691306063588601249, -0.7431448254773928008, 0.000000000000000000 ) ) ;
#8287=FACE_OUTER_BOUND ( 'NONE', #3909, .T. ) ;
#8288=ORIENTED_EDGE ( 'NONE', *, *, #1876, .F. ) ;
#8322=CIRCLE ( 'NONE', #5779, 59.51479730733485951 ) ;
#8346=EDGE_LOOP ( 'NONE', ( #768, #4298, #7696, #562 ) ) ;
#8419=CARTESIAN_POINT ( 'NONE',  ( -136.5544011653988719, 255.8380805272360590, 1.057583169244835033E-15 ) ) ;
#8421=CIRCLE ( 'NONE', #7077, 4.982234098198590644 ) ;
#8429=DIRECTION ( 'NONE',  ( -0.6691306063588565722, -0.7431448254773957984, 0.000000000000000000 ) ) ;
#8435=CIRCLE ( 'NONE', #4201, 7.000000000000016875 ) ;
#8449=EDGE_CURVE ( 'NONE', #6648, #6524, #7683, .T. ) ;
#8464=EDGE_CURVE ( 'NONE', #4542, #9316, #2084, .T. ) ;
#8498=CARTESIAN_POINT ( 'NONE',  ( -144.3499457102809913, 273.6050080517225638, 2.035728505737848743E-15 ) ) ;
#8499=DIRECTION ( 'NONE',  ( 0.000000000000000000, -1.000000000000000000, -9.100899318238108411E-17 ) ) ;
#8527=EDGE_CURVE ( 'NONE', #2342, #6087, #2772, .T. ) ;
#8531=AXIS2_PLACEMENT_3D ( 'NONE', #576, #3866, #3916 ) ;
#8538=ADVANCED_FACE ( 'NONE', ( #2959 ), #2271, .F. ) ;
#8546=DIRECTION ( 'NONE',  ( 0.000000000000000000, -1.000000000000000000, -9.100899318238108411E-17 ) ) ;
#8555=ORIENTED_EDGE ( 'NONE', *, *, #1124, .F. ) ;
#8586=CARTESIAN_POINT ( 'NONE',  ( 0.000000000000000000, 0.000000000000000000, 0.000000000000000000 ) ) ;
#8592=ORIENTED_EDGE ( 'NONE', *, *, #8464, .T. ) ;
#8645=ORIENTED_EDGE ( 'NONE', *, *, #5271, .T. ) ;
#8678=CARTESIAN_POINT ( 'NONE',  ( -43.21545076107636874, 261.9011211458127377, 9.258022131055327982E-15 ) ) ;
#8692=DIRECTION ( 'NONE',  ( -0.6691306063588565722, -0.7431448254773957984, 0.000000000000000000 ) ) ;
#8702=AXIS2_PLACEMENT_3D ( 'NONE', #9482, #9539, #7940 ) ;
#8720=AXIS2_PLACEMENT_3D ( 'NONE', #4967, #213, #1638 ) ;
#8751=AXIS2_PLACEMENT_3D ( 'NONE', #4856, #8945, #8891 ) ;
#8753=AXIS2_PLACEMENT_3D ( 'NONE', #8970, #1601, #14 ) ;
#8783=AXIS2_PLACEMENT_3D ( 'NONE', #9301, #2935, #2829 ) ;
#8792=ORIENTED_EDGE ( 'NONE', *, *, #7178, .T. ) ;
#8796=CARTESIAN_POINT ( 'NONE',  ( -93.70792096198771048, 212.3425490925494046, 6.101477040961701944E-16 ) ) ;
#8801=CARTESIAN_POINT ( 'NONE',  ( -142.3328939341254795, 249.4204141414382434, 0.000000000000000000 ) ) ;
#8809=FACE_OUTER_BOUND ( 'NONE', #8132, .T. ) ;
#8852=ORIENTED_EDGE ( 'NONE', *, *, #357, .F. ) ;
#8859=DIRECTION ( 'NONE',  ( -0.7431448254773957984, 0.6691306063588565722, -0.000000000000000000 ) ) ;
#8864=FACE_BOUND ( 'NONE', #3262, .T. ) ;
#8867=EDGE_LOOP ( 'NONE', ( #2604, #3155, #2733, #1092 ) ) ;
#8887=DIRECTION ( 'NONE',  ( -8.194486552889013533E-17, -9.100899318238110877E-17, 1.000000000000000000 ) ) ;
#8891=DIRECTION ( 'NONE',  ( -1.000000000000000000, 0.000000000000000000, 0.000000000000000000 ) ) ;
#8916=AXIS2_PLACEMENT_3D ( 'NONE', #1702, #1655, #7432 ) ;
#8917=VERTEX_POINT ( 'NONE', #3150 ) ;
#8938=FACE_OUTER_BOUND ( 'NONE', #9104, .T. ) ;
#8945=DIRECTION ( 'NONE',  ( 0.000000000000000000, -0.000000000000000000, -1.000000000000000000 ) ) ;
#8946=AXIS2_PLACEMENT_3D ( 'NONE', #3053, #6282, #7091 ) ;
#8965=EDGE_CURVE ( 'NONE', #2439, #2209, #4975, .T. ) ;
#8970=CARTESIAN_POINT ( 'NONE',  ( -122.5292777575814114, 231.5891580443559121, 0.000000000000000000 ) ) ;
#9012=ORIENTED_EDGE ( 'NONE', *, *, #2153, .T. ) ;
#9054=CARTESIAN_POINT ( 'NONE',  ( -93.80004353141508489, 205.7212393575359783, 0.000000000000000000 ) ) ;
#9073=UNCERTAINTY_MEASURE_WITH_UNIT (LENGTH_MEASURE( 1.000000000000000082E-05 ), #3530, 'distance_accuracy_value', 'NONE');
#9094=EDGE_CURVE ( 'NONE', #6578, #2209, #5318, .T. ) ;
#9095=ADVANCED_FACE ( 'NONE', ( #8287 ), #5313, .T. ) ;
#9104=EDGE_LOOP ( 'NONE', ( #5822, #7237, #1544, #9782 ) ) ;
#9107=DIRECTION ( 'NONE',  ( -1.000000000000000000, 0.000000000000000000, 0.000000000000000000 ) ) ;
#9111=ADVANCED_FACE ( 'NONE', ( #4258 ), #4803, .F. ) ;
#9120=AXIS2_PLACEMENT_3D ( 'NONE', #4146, #8170, #10461 ) ;
#9137=ORIENTED_EDGE ( 'NONE', *, *, #430, .F. ) ;
#9163=STYLED_ITEM('',(#10525),#9837);
#9173=LINE ( 'NONE', #1062, #1818 ) ;
#9229=DIRECTION ( 'NONE',  ( 0.000000000000000000, -1.000000000000000000, -9.100899318238115807E-17 ) ) ;
#9238=FACE_OUTER_BOUND ( 'NONE', #8867, .T. ) ;
#9241=DIRECTION ( 'NONE',  ( -0.6691306063588561281, -0.7431448254773960205, 0.000000000000000000 ) ) ;
#9273=EDGE_LOOP ( 'NONE', ( #2839, #1607, #5372, #9137 ) ) ;
#9277=ADVANCED_FACE ( 'NONE', ( #9662 ), #6000, .F. ) ;
#9278=DIRECTION ( 'NONE',  ( 0.000000000000000000, -0.000000000000000000, -1.000000000000000000 ) ) ;
#9289=CIRCLE ( 'NONE', #4391, 2.515249034521771510 ) ;
#9294=EDGE_CURVE ( 'NONE', #6087, #2209, #1441, .T. ) ;
#9301=CARTESIAN_POINT ( 'NONE',  ( -155.4728935706336301, 261.2517229562222951, 0.000000000000000000 ) ) ;
#9313=CARTESIAN_POINT ( 'NONE',  ( -159.2094387399987738, 254.1279851649838122, 0.000000000000000000 ) ) ;
#9316=VERTEX_POINT ( 'NONE', #7060 ) ;
#9319=EDGE_LOOP ( 'NONE', ( #3583, #3933, #1617, #9405 ) ) ;
#9348=AXIS2_PLACEMENT_3D ( 'NONE', #5333, #6480, #3009 ) ;
#9364=AXIS2_PLACEMENT_3D ( 'NONE', #7586, #4509, #8429 ) ;
#9367=EDGE_LOOP ( 'NONE', ( #5712, #1151, #9879, #585 ) ) ;
#9382=DIRECTION ( 'NONE',  ( -0.7431448254773957984, 0.6691306063588565722, -0.000000000000000000 ) ) ;
#9394=ORIENTED_EDGE ( 'NONE', *, *, #4372, .F. ) ;
#9405=ORIENTED_EDGE ( 'NONE', *, *, #8527, .F. ) ;
#9433=CARTESIAN_POINT ( 'NONE',  ( -144.3846363017538010, 149.5413575692592474, 0.000000000000000000 ) ) ;
#9440=FACE_OUTER_BOUND ( 'NONE', #8346, .T. ) ;
#9451=EDGE_LOOP ( 'NONE', ( #10294, #4490, #1813, #5663 ) ) ;
#9461=EDGE_CURVE ( 'NONE', #5603, #4450, #5932, .T. ) ;
#9473=ORIENTED_EDGE ( 'NONE', *, *, #2944, .F. ) ;
#9482=CARTESIAN_POINT ( 'NONE',  ( -136.0474385147828116, 266.3109523634597622, 0.000000000000000000 ) ) ;
#9493=DIRECTION ( 'NONE',  ( -1.000000000000000000, 0.000000000000000000, 0.000000000000000000 ) ) ;
#9517=EDGE_CURVE ( 'NONE', #6524, #6151, #2041, .T. ) ;
#9539=DIRECTION ( 'NONE',  ( 0.000000000000000000, -0.000000000000000000, -1.000000000000000000 ) ) ;
#9540=DIRECTION ( 'NONE',  ( 0.000000000000000000, -1.000000000000000000, -9.100899318238110877E-17 ) ) ;
#9541=AXIS2_PLACEMENT_3D ( 'NONE', #2346, #702, #3088 ) ;
#9559=( GEOMETRIC_REPRESENTATION_CONTEXT ( 3 ) GLOBAL_UNCERTAINTY_ASSIGNED_CONTEXT ( ( #9073 ) ) GLOBAL_UNIT_ASSIGNED_CONTEXT ( ( #3530, #2724, #6706 ) ) REPRESENTATION_CONTEXT ( 'NONE', 'WORKASPACE' ) );
#9565=DIRECTION ( 'NONE',  ( -0.6691306063588553510, -0.7431448254773969087, 0.000000000000000000 ) ) ;
#9585=EDGE_LOOP ( 'NONE', ( #1629, #9012, #3473, #3392 ) ) ;
#9596=DIRECTION ( 'NONE',  ( -0.7431448254773957984, 0.6691306063588565722, -0.000000000000000000 ) ) ;
#9602=AXIS2_PLACEMENT_3D ( 'NONE', #6400, #8142, #3809 ) ;
#9613=ORIENTED_EDGE ( 'NONE', *, *, #556, .F. ) ;
#9633=CARTESIAN_POINT ( 'NONE',  ( -136.1699968855118357, 255.5531976154833274, 1.063156219295426707E-15 ) ) ;
#9644=CIRCLE ( 'NONE', #5052, 7.572730065532343069 ) ;
#9662=FACE_OUTER_BOUND ( 'NONE', #7216, .T. ) ;
#9697=SHAPE_REPRESENTATION ( 'Plastic Grip', ( #4601 ), #9559 ) ;
#9703=AXIS2_PLACEMENT_3D ( 'NONE', #6158, #4522, #1184 ) ;
#9724=ORIENTED_EDGE ( 'NONE', *, *, #833, .F. ) ;
#9744=CARTESIAN_POINT ( 'NONE',  ( -164.8502026021585607, 257.7787449950629934, 0.000000000000000000 ) ) ;
#9745=ADVANCED_BREP_SHAPE_REPRESENTATION ( '', ( #9837, #4601 ), #9559 ) ;
#9749=AXIS2_PLACEMENT_3D ( 'NONE', #7101, #1424, #1531 ) ;
#9754=FACE_OUTER_BOUND ( 'NONE', #9319, .T. ) ;
#9756=CIRCLE ( 'NONE', #9933, 8.855570079111213744 ) ;
#9760=TOROIDAL_SURFACE ( 'NONE', #1281, -39.11828581851394659, 47.56532671630426989 ) ;
#9782=ORIENTED_EDGE ( 'NONE', *, *, #2944, .T. ) ;
#9814=DIRECTION ( 'NONE',  ( 0.000000000000000000, -0.000000000000000000, -1.000000000000000000 ) ) ;
#9831=CARTESIAN_POINT ( 'NONE',  ( -97.04168628513711781, 208.6400276031560566, 0.000000000000000000 ) ) ;
#9837=MANIFOLD_SOLID_BREP ( 'Revolve1', #7236 ) ;
#9879=ORIENTED_EDGE ( 'NONE', *, *, #101, .T. ) ;
#9888=CARTESIAN_POINT ( 'NONE',  ( -101.9861939659648726, 222.5115114232797282, 8.572527594031516577E-16 ) ) ;
#9896=ORIENTED_EDGE ( 'NONE', *, *, #9517, .T. ) ;
#9911=VERTEX_POINT ( 'NONE', #2039 ) ;
#9919=DIRECTION ( 'NONE',  ( 0.000000000000000000, -0.000000000000000000, -1.000000000000000000 ) ) ;
#9925=VERTEX_POINT ( 'NONE', #9888 ) ;
#9933=AXIS2_PLACEMENT_3D ( 'NONE', #4648, #5549, #6287 ) ;
#9979=DIRECTION ( 'NONE',  ( -1.000000000000000000, 0.000000000000000000, 0.000000000000000000 ) ) ;
#10032=AXIS2_PLACEMENT_3D ( 'NONE', #4545, #6288, #3247 ) ;
#10047=APPLICATION_CONTEXT ( 'automotive_design' ) ;
#10075=CARTESIAN_POINT ( 'NONE',  ( -97.04168628513710360, 208.6400276031560281, 0.000000000000000000 ) ) ;
#10105=CIRCLE ( 'NONE', #8751, 9.050254677131414738 ) ;
#10106=( NAMED_UNIT ( * ) SI_UNIT ( $, .STERADIAN. ) SOLID_ANGLE_UNIT ( ) );
#10125=CARTESIAN_POINT ( 'NONE',  ( -121.1992630477586346, 230.3916074206559017, 0.000000000000000000 ) ) ;
#10129=CARTESIAN_POINT ( 'NONE',  ( -94.36516385970165288, 211.6126069050656042, 4.898587196589436495E-16 ) ) ;
#10133=CIRCLE ( 'NONE', #1830, 9.050254677131414738 ) ;
#10189=EDGE_CURVE ( 'NONE', #4869, #4943, #8322, .T. ) ;
#10194=CARTESIAN_POINT ( 'NONE',  ( -134.8713710537857935, 257.7072748320279061, 1.365612337163390183E-15 ) ) ;
#10247=CARTESIAN_POINT ( 'NONE',  ( -168.7559887226706223, 267.8293446334838563, 0.000000000000000000 ) ) ;
#10281=CYLINDRICAL_SURFACE ( 'NONE', #9749, 4.000000000000016875 ) ;
#10294=ORIENTED_EDGE ( 'NONE', *, *, #6467, .T. ) ;
#10337=ORIENTED_EDGE ( 'NONE', *, *, #8449, .F. ) ;
#10403=CARTESIAN_POINT ( 'NONE',  ( -121.7299640054770578, 230.8694527092982867, 0.000000000000000000 ) ) ;
#10404=CARTESIAN_POINT ( 'NONE',  ( -142.3328939341254795, 249.4204141414382434, 0.000000000000000000 ) ) ;
#10413=AXIS2_PLACEMENT_3D ( 'NONE', #8149, #9919, #5869 ) ;
#10417=CIRCLE ( 'NONE', #1452, 70.74985237403969052 ) ;
#10437=EDGE_LOOP ( 'NONE', ( #7433, #5240, #5293, #10337 ) ) ;
#10438=DIRECTION ( 'NONE',  ( -0.7431448254773957984, 0.6691306063588565722, -0.000000000000000000 ) ) ;
#10440=EDGE_LOOP ( 'NONE', ( #5591, #5168, #4882, #1770 ) ) ;
#10461=DIRECTION ( 'NONE',  ( -0.6691306063588564612, -0.7431448254773956874, 0.000000000000000000 ) ) ;
#10519=COLOUR_RGB('Black',0.12,0.14,0.17);
#10520=FILL_AREA_STYLE_COLOUR('',#10519);
#10521=FILL_AREA_STYLE('',(#10520));
#10522=SURFACE_STYLE_FILL_AREA(#10521);
#10523=SURFACE_SIDE_STYLE('',(#10522));
#10524=SURFACE_STYLE_USAGE(.BOTH.,#10523);
#10525=PRESENTATION_STYLE_ASSIGNMENT((#10524));
ENDSEC;
END-ISO-10303-21;
